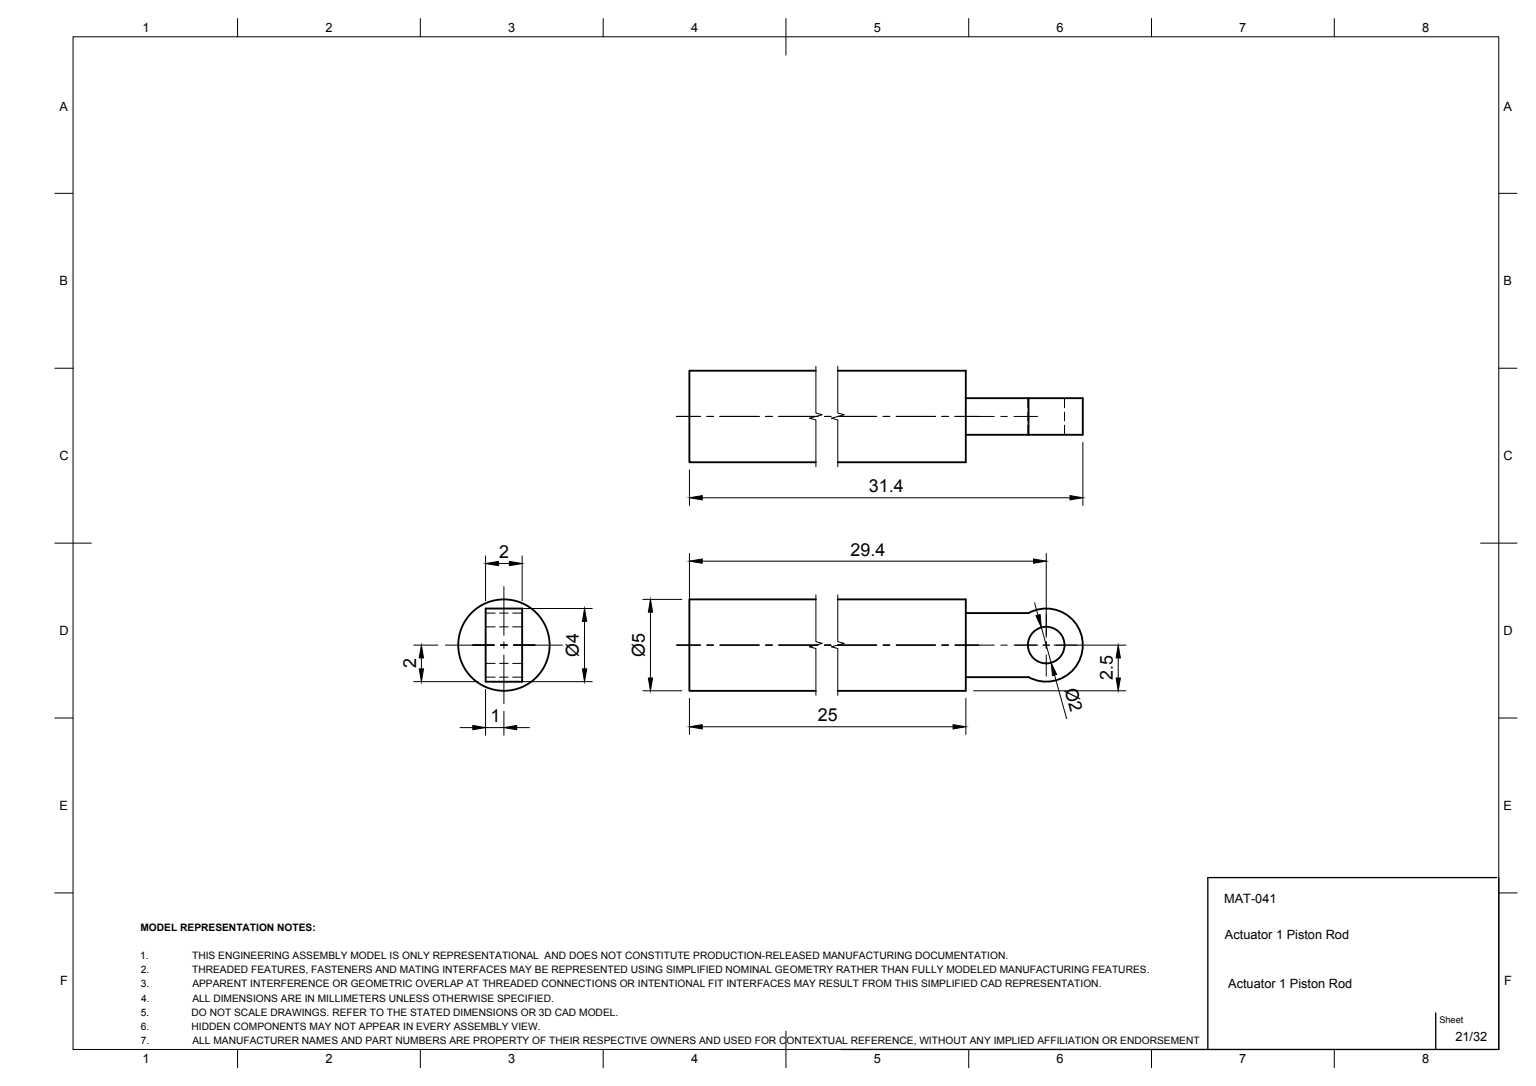
ISO-10303-21;
HEADER;
/* Generated by software containing ST-Developer
 * from STEP Tools, Inc. (www.steptools.com) 
 */

FILE_DESCRIPTION(
/* description */ ('STEP AP214'),
/* implementation_level */ '2;1');

FILE_NAME(
/* name */ 'Actuator 1 Piston Rod.step',
/* time_stamp */ '2026-11-14T21:57:47-08:00',
/* author */ (''),
/* organization */ (''),
/* preprocessor_version */ 'ST-DEVELOPER v20.2',
/* originating_system */ 'Autodesk Translation Framework v15.17.0.0',
/* authorisation */ '');

FILE_SCHEMA (('AUTOMOTIVE_DESIGN { 1 0 10303 214 3 1 1 }'));
ENDSEC;

DATA;
#10=MECHANICAL_DESIGN_GEOMETRIC_PRESENTATION_REPRESENTATION('',(#257),#13199);
#221=SHAPE_REPRESENTATION_RELATIONSHIP('SRR','None',#13292,#239);
#239=ADVANCED_BREP_SHAPE_REPRESENTATION('',(#275),#13188);
#257=STYLED_ITEM('',(#13410),#275);
#275=MANIFOLD_SOLID_BREP('Body1',#6852);
#342=FACE_BOUND('',#2502,.T.);
#343=FACE_BOUND('',#2505,.T.);
#344=FACE_BOUND('',#2508,.T.);
#518=PLANE('',#7562);
#519=PLANE('',#7563);
#520=PLANE('',#7564);
#521=PLANE('',#7565);
#522=PLANE('',#7566);
#523=PLANE('',#7567);
#923=LINE('',#11819,#1441);
#924=LINE('',#11826,#1442);
#925=LINE('',#11829,#1443);
#926=LINE('',#11834,#1444);
#927=LINE('',#11839,#1445);
#928=LINE('',#11841,#1446);
#929=LINE('',#11843,#1447);
#930=LINE('',#11844,#1448);
#931=LINE('',#11847,#1449);
#932=LINE('',#11848,#1450);
#933=LINE('',#11850,#1451);
#934=LINE('',#11852,#1452);
#1441=VECTOR('',#9132,1.);
#1442=VECTOR('',#9139,1000.);
#1443=VECTOR('',#9142,1000.);
#1444=VECTOR('',#9147,2.50000000000001);
#1445=VECTOR('',#9152,1000.);
#1446=VECTOR('',#9153,1000.);
#1447=VECTOR('',#9154,1000.);
#1448=VECTOR('',#9155,1000.);
#1449=VECTOR('',#9160,1000.);
#1450=VECTOR('',#9161,1000.);
#1451=VECTOR('',#9164,1000.);
#1452=VECTOR('',#9167,1000.);
#1748=CYLINDRICAL_SURFACE('',#7553,1.);
#1749=CYLINDRICAL_SURFACE('',#7556,2.);
#1750=CYLINDRICAL_SURFACE('',#7559,2.50000000000001);
#2049=FACE_OUTER_BOUND('',#2498,.T.);
#2050=FACE_OUTER_BOUND('',#2499,.T.);
#2051=FACE_OUTER_BOUND('',#2500,.T.);
#2052=FACE_OUTER_BOUND('',#2501,.T.);
#2053=FACE_OUTER_BOUND('',#2503,.T.);
#2054=FACE_OUTER_BOUND('',#2504,.T.);
#2055=FACE_OUTER_BOUND('',#2506,.T.);
#2056=FACE_OUTER_BOUND('',#2507,.T.);
#2057=FACE_OUTER_BOUND('',#2509,.T.);
#2498=EDGE_LOOP('',(#5748,#5749,#5750,#5751));
#2499=EDGE_LOOP('',(#5752,#5753,#5754,#5755));
#2500=EDGE_LOOP('',(#5756,#5757,#5758,#5759));
#2501=EDGE_LOOP('',(#5760));
#2502=EDGE_LOOP('',(#5761,#5762,#5763,#5764));
#2503=EDGE_LOOP('',(#5765));
#2504=EDGE_LOOP('',(#5766,#5767,#5768,#5769));
#2505=EDGE_LOOP('',(#5770));
#2506=EDGE_LOOP('',(#5771,#5772,#5773,#5774));
#2507=EDGE_LOOP('',(#5775,#5776,#5777,#5778));
#2508=EDGE_LOOP('',(#5779));
#2509=EDGE_LOOP('',(#5780,#5781,#5782,#5783));
#2897=CIRCLE('',#7554,1.);
#2898=CIRCLE('',#7555,1.);
#2899=CIRCLE('',#7557,2.);
#2900=CIRCLE('',#7558,2.);
#2901=CIRCLE('',#7560,2.50000000000001);
#2902=CIRCLE('',#7561,2.50000000000001);
#3384=VERTEX_POINT('',#11816);
#3385=VERTEX_POINT('',#11818);
#3386=VERTEX_POINT('',#11822);
#3387=VERTEX_POINT('',#11823);
#3388=VERTEX_POINT('',#11825);
#3389=VERTEX_POINT('',#11827);
#3390=VERTEX_POINT('',#11831);
#3391=VERTEX_POINT('',#11833);
#3392=VERTEX_POINT('',#11837);
#3393=VERTEX_POINT('',#11838);
#3394=VERTEX_POINT('',#11840);
#3395=VERTEX_POINT('',#11842);
#4211=EDGE_CURVE('',#3384,#3384,#2897,.T.);
#4212=EDGE_CURVE('',#3384,#3385,#923,.T.);
#4213=EDGE_CURVE('',#3385,#3385,#2898,.T.);
#4214=EDGE_CURVE('',#3386,#3387,#2899,.T.);
#4215=EDGE_CURVE('',#3388,#3386,#924,.T.);
#4216=EDGE_CURVE('',#3389,#3388,#2900,.T.);
#4217=EDGE_CURVE('',#3387,#3389,#925,.T.);
#4218=EDGE_CURVE('',#3390,#3390,#2901,.T.);
#4219=EDGE_CURVE('',#3390,#3391,#926,.T.);
#4220=EDGE_CURVE('',#3391,#3391,#2902,.T.);
#4221=EDGE_CURVE('',#3392,#3393,#927,.T.);
#4222=EDGE_CURVE('',#3394,#3392,#928,.T.);
#4223=EDGE_CURVE('',#3395,#3394,#929,.T.);
#4224=EDGE_CURVE('',#3393,#3395,#930,.T.);
#4225=EDGE_CURVE('',#3389,#3392,#931,.T.);
#4226=EDGE_CURVE('',#3388,#3394,#932,.T.);
#4227=EDGE_CURVE('',#3387,#3393,#933,.T.);
#4228=EDGE_CURVE('',#3386,#3395,#934,.T.);
#5748=ORIENTED_EDGE('',*,*,#4211,.F.);
#5749=ORIENTED_EDGE('',*,*,#4212,.T.);
#5750=ORIENTED_EDGE('',*,*,#4213,.T.);
#5751=ORIENTED_EDGE('',*,*,#4212,.F.);
#5752=ORIENTED_EDGE('',*,*,#4214,.F.);
#5753=ORIENTED_EDGE('',*,*,#4215,.F.);
#5754=ORIENTED_EDGE('',*,*,#4216,.F.);
#5755=ORIENTED_EDGE('',*,*,#4217,.F.);
#5756=ORIENTED_EDGE('',*,*,#4218,.T.);
#5757=ORIENTED_EDGE('',*,*,#4219,.T.);
#5758=ORIENTED_EDGE('',*,*,#4220,.F.);
#5759=ORIENTED_EDGE('',*,*,#4219,.F.);
#5760=ORIENTED_EDGE('',*,*,#4220,.T.);
#5761=ORIENTED_EDGE('',*,*,#4221,.F.);
#5762=ORIENTED_EDGE('',*,*,#4222,.F.);
#5763=ORIENTED_EDGE('',*,*,#4223,.F.);
#5764=ORIENTED_EDGE('',*,*,#4224,.F.);
#5765=ORIENTED_EDGE('',*,*,#4218,.F.);
#5766=ORIENTED_EDGE('',*,*,#4225,.F.);
#5767=ORIENTED_EDGE('',*,*,#4216,.T.);
#5768=ORIENTED_EDGE('',*,*,#4226,.T.);
#5769=ORIENTED_EDGE('',*,*,#4222,.T.);
#5770=ORIENTED_EDGE('',*,*,#4213,.F.);
#5771=ORIENTED_EDGE('',*,*,#4227,.F.);
#5772=ORIENTED_EDGE('',*,*,#4217,.T.);
#5773=ORIENTED_EDGE('',*,*,#4225,.T.);
#5774=ORIENTED_EDGE('',*,*,#4221,.T.);
#5775=ORIENTED_EDGE('',*,*,#4214,.T.);
#5776=ORIENTED_EDGE('',*,*,#4227,.T.);
#5777=ORIENTED_EDGE('',*,*,#4224,.T.);
#5778=ORIENTED_EDGE('',*,*,#4228,.F.);
#5779=ORIENTED_EDGE('',*,*,#4211,.T.);
#5780=ORIENTED_EDGE('',*,*,#4226,.F.);
#5781=ORIENTED_EDGE('',*,*,#4215,.T.);
#5782=ORIENTED_EDGE('',*,*,#4228,.T.);
#5783=ORIENTED_EDGE('',*,*,#4223,.T.);
#6701=ADVANCED_FACE('',(#2049),#1748,.F.);
#6702=ADVANCED_FACE('',(#2050),#1749,.T.);
#6703=ADVANCED_FACE('',(#2051),#1750,.T.);
#6704=ADVANCED_FACE('',(#2052,#342),#518,.T.);
#6705=ADVANCED_FACE('',(#2053),#519,.F.);
#6706=ADVANCED_FACE('',(#2054,#343),#520,.F.);
#6707=ADVANCED_FACE('',(#2055),#521,.F.);
#6708=ADVANCED_FACE('',(#2056,#344),#522,.F.);
#6709=ADVANCED_FACE('',(#2057),#523,.F.);
#6852=CLOSED_SHELL('',(#6701,#6702,#6703,#6704,#6705,#6706,#6707,#6708,
#6709));
#7552=AXIS2_PLACEMENT_3D('',#11814,#9126,#9127);
#7553=AXIS2_PLACEMENT_3D('',#11815,#9128,#9129);
#7554=AXIS2_PLACEMENT_3D('',#11817,#9130,#9131);
#7555=AXIS2_PLACEMENT_3D('',#11820,#9133,#9134);
#7556=AXIS2_PLACEMENT_3D('',#11821,#9135,#9136);
#7557=AXIS2_PLACEMENT_3D('',#11824,#9137,#9138);
#7558=AXIS2_PLACEMENT_3D('',#11828,#9140,#9141);
#7559=AXIS2_PLACEMENT_3D('',#11830,#9143,#9144);
#7560=AXIS2_PLACEMENT_3D('',#11832,#9145,#9146);
#7561=AXIS2_PLACEMENT_3D('',#11835,#9148,#9149);
#7562=AXIS2_PLACEMENT_3D('',#11836,#9150,#9151);
#7563=AXIS2_PLACEMENT_3D('',#11845,#9156,#9157);
#7564=AXIS2_PLACEMENT_3D('',#11846,#9158,#9159);
#7565=AXIS2_PLACEMENT_3D('',#11849,#9162,#9163);
#7566=AXIS2_PLACEMENT_3D('',#11851,#9165,#9166);
#7567=AXIS2_PLACEMENT_3D('',#11853,#9168,#9169);
#9126=DIRECTION('axis',(0.,0.,1.));
#9127=DIRECTION('refdir',(1.,0.,0.));
#9128=DIRECTION('center_axis',(1.,1.23908819712629E-16,0.));
#9129=DIRECTION('ref_axis',(-1.23908819712629E-16,1.,0.));
#9130=DIRECTION('center_axis',(1.,1.23908819712629E-16,0.));
#9131=DIRECTION('ref_axis',(-1.23908819712629E-16,1.,0.));
#9132=DIRECTION('',(1.,1.23908819712629E-16,0.));
#9133=DIRECTION('center_axis',(1.,1.23908819712629E-16,0.));
#9134=DIRECTION('ref_axis',(-1.23908819712629E-16,1.,0.));
#9135=DIRECTION('center_axis',(1.,1.23908819712629E-16,0.));
#9136=DIRECTION('ref_axis',(-1.54074395550979E-32,6.12323399573677E-17,
1.));
#9137=DIRECTION('center_axis',(-1.,-1.23908819712629E-16,0.));
#9138=DIRECTION('ref_axis',(-1.23908819712629E-16,1.,0.));
#9139=DIRECTION('',(-1.,-1.23908819712629E-16,0.));
#9140=DIRECTION('center_axis',(1.,1.23908819712629E-16,0.));
#9141=DIRECTION('ref_axis',(-1.23908819712629E-16,1.,0.));
#9142=DIRECTION('',(1.,1.23908819712629E-16,0.));
#9143=DIRECTION('center_axis',(0.,0.,-1.));
#9144=DIRECTION('ref_axis',(-1.,-4.93038065763131E-32,0.));
#9145=DIRECTION('center_axis',(0.,0.,1.));
#9146=DIRECTION('ref_axis',(1.,4.93038065763131E-32,0.));
#9147=DIRECTION('',(0.,0.,1.));
#9148=DIRECTION('center_axis',(0.,0.,1.));
#9149=DIRECTION('ref_axis',(1.,4.93038065763131E-32,0.));
#9150=DIRECTION('center_axis',(0.,0.,1.));
#9151=DIRECTION('ref_axis',(1.,4.93038065763131E-32,0.));
#9152=DIRECTION('',(-1.,-4.93038065763131E-32,0.));
#9153=DIRECTION('',(-1.23908819712629E-16,1.,0.));
#9154=DIRECTION('',(1.,4.93038065763131E-32,0.));
#9155=DIRECTION('',(1.23908819712629E-16,-1.,0.));
#9156=DIRECTION('center_axis',(0.,0.,1.));
#9157=DIRECTION('ref_axis',(1.,4.93038065763131E-32,0.));
#9158=DIRECTION('center_axis',(-1.,-1.23908819712629E-16,0.));
#9159=DIRECTION('ref_axis',(1.23908819712629E-16,-1.,0.));
#9160=DIRECTION('',(0.,0.,-1.));
#9161=DIRECTION('',(0.,0.,-1.));
#9162=DIRECTION('center_axis',(4.93038065763131E-32,-1.,0.));
#9163=DIRECTION('ref_axis',(0.,0.,-1.));
#9164=DIRECTION('',(0.,0.,-1.));
#9165=DIRECTION('center_axis',(1.,1.23908819712629E-16,0.));
#9166=DIRECTION('ref_axis',(-1.23908819712629E-16,1.,0.));
#9167=DIRECTION('',(0.,0.,-1.));
#9168=DIRECTION('center_axis',(-4.93038065763131E-32,1.,0.));
#9169=DIRECTION('ref_axis',(0.,0.,1.));
#11814=CARTESIAN_POINT('',(0.,0.,0.));
#11815=CARTESIAN_POINT('Origin',(-1.,-6.50521303491303E-16,29.4));
#11816=CARTESIAN_POINT('',(-1.,-1.,29.4));
#11817=CARTESIAN_POINT('Origin',(-1.,-6.50521303491303E-16,29.4));
#11818=CARTESIAN_POINT('',(1.00000000000001,-1.,29.4));
#11819=CARTESIAN_POINT('',(-1.,-1.,29.4));
#11820=CARTESIAN_POINT('Origin',(1.00000000000001,-4.33680868994202E-16,
29.4));
#11821=CARTESIAN_POINT('Origin',(-6.6568542494924,-2.16840434497101E-16,
29.4));
#11822=CARTESIAN_POINT('',(-1.,-1.75000000000001,28.4317541634482));
#11823=CARTESIAN_POINT('',(-1.,1.75000000000001,28.4317541634482));
#11824=CARTESIAN_POINT('Origin',(-1.,-6.50521303491303E-16,29.4));
#11825=CARTESIAN_POINT('',(1.,-1.75000000000001,28.4317541634482));
#11826=CARTESIAN_POINT('',(-6.6568542494924,-1.75,28.4317541634482));
#11827=CARTESIAN_POINT('',(1.,1.75000000000001,28.4317541634482));
#11828=CARTESIAN_POINT('Origin',(1.00000000000001,-4.33680868994202E-16,
29.4));
#11829=CARTESIAN_POINT('',(-6.65685424949239,1.75000000000001,28.4317541634482));
#11830=CARTESIAN_POINT('Origin',(0.,0.,25.));
#11831=CARTESIAN_POINT('',(2.50000000000001,-3.06161699786839E-16,0.));
#11832=CARTESIAN_POINT('Origin',(0.,0.,0.));
#11833=CARTESIAN_POINT('',(2.50000000000001,-3.06161699786839E-16,25.));
#11834=CARTESIAN_POINT('',(2.50000000000001,-3.06161699786839E-16,25.));
#11835=CARTESIAN_POINT('Origin',(0.,0.,25.));
#11836=CARTESIAN_POINT('Origin',(0.,0.,25.));
#11837=CARTESIAN_POINT('',(1.,1.75000000000001,25.));
#11838=CARTESIAN_POINT('',(-1.,1.75000000000001,25.));
#11839=CARTESIAN_POINT('',(-1.,1.75000000000001,25.));
#11840=CARTESIAN_POINT('',(1.,-1.75000000000001,25.));
#11841=CARTESIAN_POINT('',(1.,1.75000000000001,25.));
#11842=CARTESIAN_POINT('',(-1.,-1.75000000000001,25.));
#11843=CARTESIAN_POINT('',(-1.,-1.75000000000001,25.));
#11844=CARTESIAN_POINT('',(-1.,1.75000000000001,25.));
#11845=CARTESIAN_POINT('Origin',(0.,0.,0.));
#11846=CARTESIAN_POINT('Origin',(1.,1.75000000000001,29.4));
#11847=CARTESIAN_POINT('',(1.,1.75000000000001,29.4));
#11848=CARTESIAN_POINT('',(1.,-1.75000000000001,29.4));
#11849=CARTESIAN_POINT('Origin',(-1.,1.75000000000001,29.4));
#11850=CARTESIAN_POINT('',(-1.,1.75000000000001,29.4));
#11851=CARTESIAN_POINT('Origin',(-1.,1.75000000000001,29.4));
#11852=CARTESIAN_POINT('',(-1.,-1.75000000000001,29.4));
#11853=CARTESIAN_POINT('Origin',(-1.,-1.75000000000001,29.4));
#13162=UNCERTAINTY_MEASURE_WITH_UNIT(LENGTH_MEASURE(0.01),#13200,
'DISTANCE_ACCURACY_VALUE',
'Maximum model space distance between geometric entities at asserted c
onnectivities');
#13173=UNCERTAINTY_MEASURE_WITH_UNIT(LENGTH_MEASURE(0.01),#13200,
'DISTANCE_ACCURACY_VALUE',
'Maximum model space distance between geometric entities at asserted c
onnectivities');
#13188=(
GEOMETRIC_REPRESENTATION_CONTEXT(3)
GLOBAL_UNCERTAINTY_ASSIGNED_CONTEXT((#13162))
GLOBAL_UNIT_ASSIGNED_CONTEXT((#13200,#13202,#13203))
REPRESENTATION_CONTEXT('','3D')
);
#13199=(
GEOMETRIC_REPRESENTATION_CONTEXT(3)
GLOBAL_UNCERTAINTY_ASSIGNED_CONTEXT((#13173))
GLOBAL_UNIT_ASSIGNED_CONTEXT((#13200,#13202,#13203))
REPRESENTATION_CONTEXT('','3D')
);
#13200=(
LENGTH_UNIT()
NAMED_UNIT(*)
SI_UNIT(.MILLI.,.METRE.)
);
#13202=(
NAMED_UNIT(*)
PLANE_ANGLE_UNIT()
SI_UNIT($,.RADIAN.)
);
#13203=(
NAMED_UNIT(*)
SI_UNIT($,.STERADIAN.)
SOLID_ANGLE_UNIT()
);
#13218=SHAPE_DEFINITION_REPRESENTATION(#13247,#13292);
#13247=PRODUCT_DEFINITION_SHAPE('',$,#13318);
#13292=SHAPE_REPRESENTATION('',(#7552),#13188);
#13303=PRODUCT_DEFINITION_CONTEXT('part definition',#13380,'design');
#13318=PRODUCT_DEFINITION('Actuator 1 Piston Rod',
'Actuator 1 Piston Rod',#13343,#13303);
#13343=PRODUCT_DEFINITION_FORMATION('',$,#13396);
#13380=APPLICATION_CONTEXT(
'Core Data for Automotive Mechanical Design Process');
#13381=PRODUCT_CONTEXT('part definition',#13380,'mechanical');
#13396=PRODUCT('Actuator 1 Piston Rod','Actuator 1 Piston Rod',$,(#13381));
#13410=PRESENTATION_STYLE_ASSIGNMENT((#13415));
#13415=SURFACE_STYLE_USAGE(.BOTH.,#13420);
#13420=SURFACE_SIDE_STYLE('',(#13425));
#13425=SURFACE_STYLE_FILL_AREA(#13430);
#13430=FILL_AREA_STYLE('Opaque(227,224,212)',(#13435));
#13435=FILL_AREA_STYLE_COLOUR('Opaque(227,224,212)',#13440);
#13440=COLOUR_RGB('Opaque(227,224,212)',0.890196078431372,0.87843137254902,
0.831372549019608);
ENDSEC;
END-ISO-10303-21;
